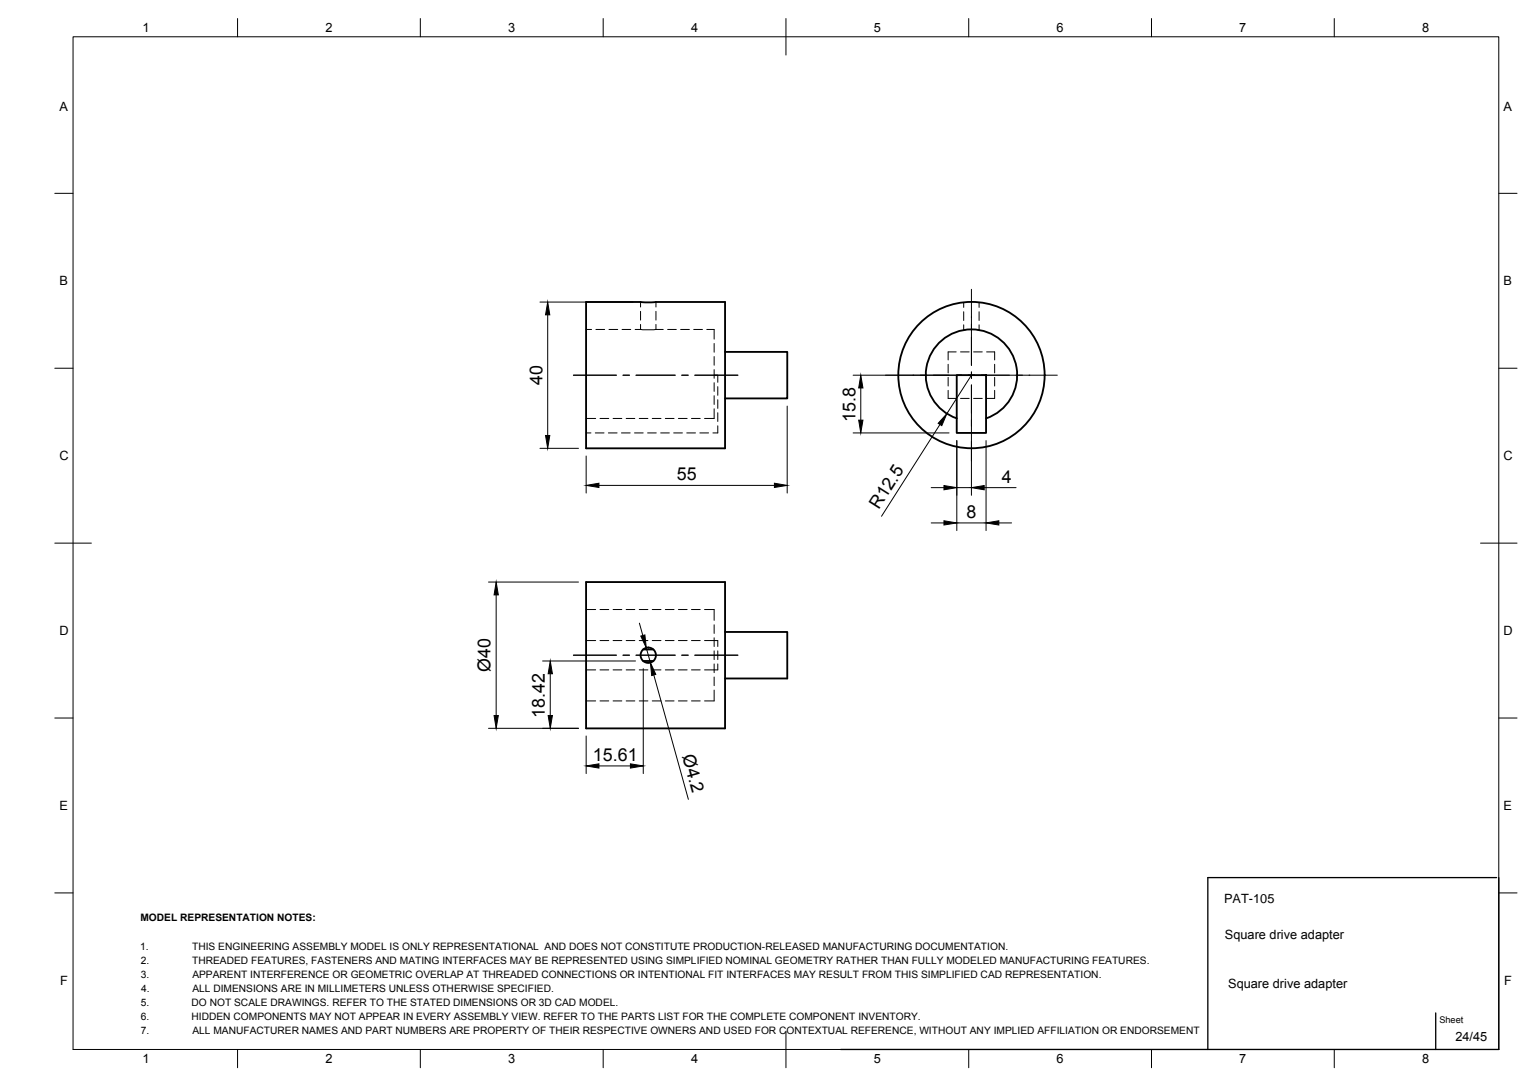
ISO-10303-21;
HEADER;
/* Generated by software containing ST-Developer
 * from STEP Tools, Inc. (www.steptools.com) 
 */

FILE_DESCRIPTION(
/* description */ ('Torque wrench calibration arm'),
/* implementation_level */ '2;1');

FILE_NAME(
/* name */ 'Square drive adapter.step',
/* time_stamp */ '2026-10-28T03:24:52-07:00',
/* author */ (''),
/* organization */ (''),
/* preprocessor_version */ 'ST-DEVELOPER v20.2',
/* originating_system */ 'Autodesk Translation Framework v15.17.0.0',
/* authorisation */ '');

FILE_SCHEMA (('AUTOMOTIVE_DESIGN { 1 0 10303 214 3 1 1 }'));
ENDSEC;

DATA;
#10=MECHANICAL_DESIGN_GEOMETRIC_PRESENTATION_REPRESENTATION('',(#452),#12783);
#267=B_SPLINE_CURVE_WITH_KNOTS('',3,(#11399,#11400,#11401,#11402,#11403,
#11404,#11405,#11406,#11407,#11408,#11409,#11410,#11411,#11412),
 .UNSPECIFIED.,.F.,.F.,(4,2,2,2,2,2,4),(0.779149138325151,0.792661737650614,
0.87192659943798,0.951191461225345,1.03045632301271,1.10972118480008,1.12323378412554),
 .UNSPECIFIED.);
#268=B_SPLINE_CURVE_WITH_KNOTS('',3,(#11418,#11419,#11420,#11421,#11422,
#11423,#11424,#11425,#11426,#11427,#11428,#11429,#11430,#11431,#11432,#11433,
#11434,#11435),.UNSPECIFIED.,.F.,.F.,(4,2,2,2,2,2,2,2,4),(0.,0.0791670250779304,
0.158334050155861,0.237500747381212,0.316667444606564,0.395834141831915,
0.475000839057267,0.554167864135197,0.633334889213128),.UNSPECIFIED.);
#269=B_SPLINE_CURVE_WITH_KNOTS('',3,(#11436,#11437,#11438,#11439,#11440,
#11441,#11442,#11443,#11444,#11445,#11446,#11447,#11448,#11449,#11450,#11451,
#11452,#11453),.UNSPECIFIED.,.F.,.F.,(4,2,2,2,2,2,2,2,4),(0.633334889213128,
0.712501914291058,0.791668939368988,0.87083563659434,0.950002333819691,
1.02916903104504,1.10833572827039,1.18750275334832,1.26666977842626),
 .UNSPECIFIED.);
#270=B_SPLINE_CURVE_WITH_KNOTS('',3,(#11456,#11457,#11458,#11459,#11460,
#11461,#11462,#11463,#11464,#11465,#11466,#11467,#11468,#11469),
 .UNSPECIFIED.,.F.,.F.,(4,2,2,2,2,2,4),(0.145021497508255,0.158534096833718,
0.237798958621083,0.317063820408448,0.396328682195814,0.475593543983179,
0.489106143308642),.UNSPECIFIED.);
#369=SHAPE_REPRESENTATION_RELATIONSHIP('SRR','None',#12952,#406);
#406=ADVANCED_BREP_SHAPE_REPRESENTATION('',(#504),#12761);
#452=STYLED_ITEM('',(#13198),#504);
#504=MANIFOLD_SOLID_BREP('Body1',#6523);
#604=FACE_BOUND('',#1568,.T.);
#605=FACE_BOUND('',#1576,.T.);
#606=FACE_BOUND('',#1578,.T.);
#607=FACE_BOUND('',#1580,.T.);
#770=PLANE('',#7428);
#771=PLANE('',#7433);
#772=PLANE('',#7434);
#773=PLANE('',#7435);
#774=PLANE('',#7436);
#775=PLANE('',#7437);
#776=PLANE('',#7438);
#777=PLANE('',#7439);
#778=PLANE('',#7442);
#779=PLANE('',#7443);
#780=PLANE('',#7444);
#781=PLANE('',#7445);
#782=PLANE('',#7446);
#783=PLANE('',#7447);
#784=PLANE('',#7449);
#1091=FACE_OUTER_BOUND('',#1559,.T.);
#1092=FACE_OUTER_BOUND('',#1560,.T.);
#1093=FACE_OUTER_BOUND('',#1561,.T.);
#1094=FACE_OUTER_BOUND('',#1562,.T.);
#1095=FACE_OUTER_BOUND('',#1563,.T.);
#1096=FACE_OUTER_BOUND('',#1564,.T.);
#1097=FACE_OUTER_BOUND('',#1565,.T.);
#1098=FACE_OUTER_BOUND('',#1566,.T.);
#1099=FACE_OUTER_BOUND('',#1567,.T.);
#1100=FACE_OUTER_BOUND('',#1569,.T.);
#1101=FACE_OUTER_BOUND('',#1570,.T.);
#1102=FACE_OUTER_BOUND('',#1571,.T.);
#1103=FACE_OUTER_BOUND('',#1572,.T.);
#1104=FACE_OUTER_BOUND('',#1573,.T.);
#1105=FACE_OUTER_BOUND('',#1574,.T.);
#1106=FACE_OUTER_BOUND('',#1575,.T.);
#1107=FACE_OUTER_BOUND('',#1577,.T.);
#1108=FACE_OUTER_BOUND('',#1579,.T.);
#1559=EDGE_LOOP('',(#5259,#5260));
#1560=EDGE_LOOP('',(#5261,#5262,#5263,#5264,#5265,#5266,#5267,#5268,#5269));
#1561=EDGE_LOOP('',(#5270,#5271,#5272));
#1562=EDGE_LOOP('',(#5273,#5274,#5275,#5276));
#1563=EDGE_LOOP('',(#5277,#5278,#5279,#5280,#5281,#5282));
#1564=EDGE_LOOP('',(#5283,#5284,#5285,#5286,#5287,#5288));
#1565=EDGE_LOOP('',(#5289,#5290,#5291,#5292));
#1566=EDGE_LOOP('',(#5293,#5294,#5295,#5296));
#1567=EDGE_LOOP('',(#5297));
#1568=EDGE_LOOP('',(#5298,#5299,#5300,#5301));
#1569=EDGE_LOOP('',(#5302,#5303,#5304,#5305));
#1570=EDGE_LOOP('',(#5306,#5307,#5308,#5309));
#1571=EDGE_LOOP('',(#5310,#5311,#5312,#5313));
#1572=EDGE_LOOP('',(#5314,#5315,#5316,#5317));
#1573=EDGE_LOOP('',(#5318,#5319,#5320,#5321));
#1574=EDGE_LOOP('',(#5322,#5323,#5324,#5325));
#1575=EDGE_LOOP('',(#5326));
#1576=EDGE_LOOP('',(#5327,#5328,#5329,#5330));
#1577=EDGE_LOOP('',(#5331,#5332,#5333,#5334));
#1578=EDGE_LOOP('',(#5335,#5336,#5337,#5338));
#1579=EDGE_LOOP('',(#5339,#5340,#5341,#5342));
#1580=EDGE_LOOP('',(#5343,#5344));
#2014=LINE('',#11395,#2429);
#2015=LINE('',#11416,#2430);
#2016=LINE('',#11471,#2431);
#2017=LINE('',#11475,#2432);
#2018=LINE('',#11477,#2433);
#2019=LINE('',#11479,#2434);
#2020=LINE('',#11480,#2435);
#2021=LINE('',#11483,#2436);
#2022=LINE('',#11485,#2437);
#2023=LINE('',#11487,#2438);
#2024=LINE('',#11489,#2439);
#2025=LINE('',#11490,#2440);
#2026=LINE('',#11493,#2441);
#2027=LINE('',#11495,#2442);
#2028=LINE('',#11497,#2443);
#2029=LINE('',#11499,#2444);
#2030=LINE('',#11500,#2445);
#2031=LINE('',#11502,#2446);
#2032=LINE('',#11503,#2447);
#2033=LINE('',#11512,#2448);
#2034=LINE('',#11514,#2449);
#2035=LINE('',#11516,#2450);
#2036=LINE('',#11517,#2451);
#2037=LINE('',#11520,#2452);
#2038=LINE('',#11522,#2453);
#2039=LINE('',#11523,#2454);
#2040=LINE('',#11526,#2455);
#2041=LINE('',#11528,#2456);
#2042=LINE('',#11529,#2457);
#2043=LINE('',#11531,#2458);
#2044=LINE('',#11532,#2459);
#2045=LINE('',#11541,#2460);
#2429=VECTOR('',#8976,1.);
#2430=VECTOR('',#8983,0.21);
#2431=VECTOR('',#8988,1.);
#2432=VECTOR('',#8991,1.);
#2433=VECTOR('',#8992,1.);
#2434=VECTOR('',#8993,1.);
#2435=VECTOR('',#8994,1.);
#2436=VECTOR('',#8997,1.);
#2437=VECTOR('',#8998,1.);
#2438=VECTOR('',#8999,1.);
#2439=VECTOR('',#9000,1.);
#2440=VECTOR('',#9001,1.);
#2441=VECTOR('',#9004,1.);
#2442=VECTOR('',#9005,1.);
#2443=VECTOR('',#9006,1.);
#2444=VECTOR('',#9007,1.);
#2445=VECTOR('',#9008,1.);
#2446=VECTOR('',#9011,1.);
#2447=VECTOR('',#9012,1.);
#2448=VECTOR('',#9023,1.);
#2449=VECTOR('',#9024,1.);
#2450=VECTOR('',#9025,1.);
#2451=VECTOR('',#9026,1.);
#2452=VECTOR('',#9029,1.);
#2453=VECTOR('',#9030,1.);
#2454=VECTOR('',#9031,1.);
#2455=VECTOR('',#9034,1.);
#2456=VECTOR('',#9035,1.);
#2457=VECTOR('',#9036,1.);
#2458=VECTOR('',#9039,1.);
#2459=VECTOR('',#9040,1.);
#2460=VECTOR('',#9055,2.);
#2820=CIRCLE('',#7429,0.21);
#2821=CIRCLE('',#7431,0.21);
#2822=CIRCLE('',#7432,0.21);
#2823=CIRCLE('',#7440,2.);
#2824=CIRCLE('',#7441,1.25);
#2825=CIRCLE('',#7448,1.25);
#2826=CIRCLE('',#7450,2.);
#3282=VERTEX_POINT('',#11393);
#3283=VERTEX_POINT('',#11394);
#3284=VERTEX_POINT('',#11398);
#3285=VERTEX_POINT('',#11413);
#3286=VERTEX_POINT('',#11415);
#3287=VERTEX_POINT('',#11417);
#3288=VERTEX_POINT('',#11454);
#3289=VERTEX_POINT('',#11473);
#3290=VERTEX_POINT('',#11474);
#3291=VERTEX_POINT('',#11476);
#3292=VERTEX_POINT('',#11478);
#3293=VERTEX_POINT('',#11482);
#3294=VERTEX_POINT('',#11484);
#3295=VERTEX_POINT('',#11486);
#3296=VERTEX_POINT('',#11488);
#3297=VERTEX_POINT('',#11492);
#3298=VERTEX_POINT('',#11494);
#3299=VERTEX_POINT('',#11496);
#3300=VERTEX_POINT('',#11498);
#3301=VERTEX_POINT('',#11506);
#3302=VERTEX_POINT('',#11510);
#3303=VERTEX_POINT('',#11511);
#3304=VERTEX_POINT('',#11513);
#3305=VERTEX_POINT('',#11515);
#3306=VERTEX_POINT('',#11519);
#3307=VERTEX_POINT('',#11521);
#3308=VERTEX_POINT('',#11525);
#3309=VERTEX_POINT('',#11527);
#3310=VERTEX_POINT('',#11537);
#3987=EDGE_CURVE('',#3282,#3283,#2014,.T.);
#3988=EDGE_CURVE('',#3282,#3283,#2820,.T.);
#3989=EDGE_CURVE('',#3284,#3282,#267,.T.);
#3990=EDGE_CURVE('',#3285,#3284,#2821,.T.);
#3991=EDGE_CURVE('',#3285,#3286,#2015,.T.);
#3992=EDGE_CURVE('',#3287,#3286,#268,.T.);
#3993=EDGE_CURVE('',#3286,#3287,#269,.T.);
#3994=EDGE_CURVE('',#3288,#3285,#2822,.T.);
#3995=EDGE_CURVE('',#3283,#3288,#270,.T.);
#3996=EDGE_CURVE('',#3288,#3284,#2016,.T.);
#3997=EDGE_CURVE('',#3289,#3290,#2017,.T.);
#3998=EDGE_CURVE('',#3291,#3289,#2018,.T.);
#3999=EDGE_CURVE('',#3291,#3292,#2019,.T.);
#4000=EDGE_CURVE('',#3292,#3290,#2020,.T.);
#4001=EDGE_CURVE('',#3290,#3293,#2021,.T.);
#4002=EDGE_CURVE('',#3292,#3294,#2022,.T.);
#4003=EDGE_CURVE('',#3294,#3295,#2023,.T.);
#4004=EDGE_CURVE('',#3296,#3295,#2024,.T.);
#4005=EDGE_CURVE('',#3293,#3296,#2025,.T.);
#4006=EDGE_CURVE('',#3297,#3289,#2026,.T.);
#4007=EDGE_CURVE('',#3298,#3297,#2027,.T.);
#4008=EDGE_CURVE('',#3299,#3298,#2028,.T.);
#4009=EDGE_CURVE('',#3300,#3299,#2029,.T.);
#4010=EDGE_CURVE('',#3300,#3291,#2030,.T.);
#4011=EDGE_CURVE('',#3295,#3299,#2031,.T.);
#4012=EDGE_CURVE('',#3294,#3300,#2032,.T.);
#4013=EDGE_CURVE('',#3301,#3301,#2823,.T.);
#4014=EDGE_CURVE('',#3293,#3297,#2824,.T.);
#4015=EDGE_CURVE('',#3302,#3303,#2033,.T.);
#4016=EDGE_CURVE('',#3302,#3304,#2034,.T.);
#4017=EDGE_CURVE('',#3305,#3304,#2035,.T.);
#4018=EDGE_CURVE('',#3303,#3305,#2036,.T.);
#4019=EDGE_CURVE('',#3303,#3306,#2037,.T.);
#4020=EDGE_CURVE('',#3307,#3305,#2038,.T.);
#4021=EDGE_CURVE('',#3306,#3307,#2039,.T.);
#4022=EDGE_CURVE('',#3306,#3308,#2040,.T.);
#4023=EDGE_CURVE('',#3309,#3307,#2041,.T.);
#4024=EDGE_CURVE('',#3308,#3309,#2042,.T.);
#4025=EDGE_CURVE('',#3308,#3302,#2043,.T.);
#4026=EDGE_CURVE('',#3304,#3309,#2044,.T.);
#4027=EDGE_CURVE('',#3296,#3298,#2825,.T.);
#4028=EDGE_CURVE('',#3310,#3310,#2826,.T.);
#4029=EDGE_CURVE('',#3301,#3310,#2045,.T.);
#5259=ORIENTED_EDGE('',*,*,#3987,.F.);
#5260=ORIENTED_EDGE('',*,*,#3988,.T.);
#5261=ORIENTED_EDGE('',*,*,#3989,.F.);
#5262=ORIENTED_EDGE('',*,*,#3990,.F.);
#5263=ORIENTED_EDGE('',*,*,#3991,.T.);
#5264=ORIENTED_EDGE('',*,*,#3992,.F.);
#5265=ORIENTED_EDGE('',*,*,#3993,.F.);
#5266=ORIENTED_EDGE('',*,*,#3991,.F.);
#5267=ORIENTED_EDGE('',*,*,#3994,.F.);
#5268=ORIENTED_EDGE('',*,*,#3995,.F.);
#5269=ORIENTED_EDGE('',*,*,#3988,.F.);
#5270=ORIENTED_EDGE('',*,*,#3996,.F.);
#5271=ORIENTED_EDGE('',*,*,#3994,.T.);
#5272=ORIENTED_EDGE('',*,*,#3990,.T.);
#5273=ORIENTED_EDGE('',*,*,#3997,.F.);
#5274=ORIENTED_EDGE('',*,*,#3998,.F.);
#5275=ORIENTED_EDGE('',*,*,#3999,.T.);
#5276=ORIENTED_EDGE('',*,*,#4000,.T.);
#5277=ORIENTED_EDGE('',*,*,#4001,.F.);
#5278=ORIENTED_EDGE('',*,*,#4000,.F.);
#5279=ORIENTED_EDGE('',*,*,#4002,.T.);
#5280=ORIENTED_EDGE('',*,*,#4003,.T.);
#5281=ORIENTED_EDGE('',*,*,#4004,.F.);
#5282=ORIENTED_EDGE('',*,*,#4005,.F.);
#5283=ORIENTED_EDGE('',*,*,#4006,.F.);
#5284=ORIENTED_EDGE('',*,*,#4007,.F.);
#5285=ORIENTED_EDGE('',*,*,#4008,.F.);
#5286=ORIENTED_EDGE('',*,*,#4009,.F.);
#5287=ORIENTED_EDGE('',*,*,#4010,.T.);
#5288=ORIENTED_EDGE('',*,*,#3998,.T.);
#5289=ORIENTED_EDGE('',*,*,#4011,.F.);
#5290=ORIENTED_EDGE('',*,*,#4003,.F.);
#5291=ORIENTED_EDGE('',*,*,#4012,.T.);
#5292=ORIENTED_EDGE('',*,*,#4009,.T.);
#5293=ORIENTED_EDGE('',*,*,#4012,.F.);
#5294=ORIENTED_EDGE('',*,*,#4002,.F.);
#5295=ORIENTED_EDGE('',*,*,#3999,.F.);
#5296=ORIENTED_EDGE('',*,*,#4010,.F.);
#5297=ORIENTED_EDGE('',*,*,#4013,.T.);
#5298=ORIENTED_EDGE('',*,*,#4006,.T.);
#5299=ORIENTED_EDGE('',*,*,#3997,.T.);
#5300=ORIENTED_EDGE('',*,*,#4001,.T.);
#5301=ORIENTED_EDGE('',*,*,#4014,.T.);
#5302=ORIENTED_EDGE('',*,*,#4015,.F.);
#5303=ORIENTED_EDGE('',*,*,#4016,.T.);
#5304=ORIENTED_EDGE('',*,*,#4017,.F.);
#5305=ORIENTED_EDGE('',*,*,#4018,.F.);
#5306=ORIENTED_EDGE('',*,*,#4019,.F.);
#5307=ORIENTED_EDGE('',*,*,#4018,.T.);
#5308=ORIENTED_EDGE('',*,*,#4020,.F.);
#5309=ORIENTED_EDGE('',*,*,#4021,.F.);
#5310=ORIENTED_EDGE('',*,*,#4022,.F.);
#5311=ORIENTED_EDGE('',*,*,#4021,.T.);
#5312=ORIENTED_EDGE('',*,*,#4023,.F.);
#5313=ORIENTED_EDGE('',*,*,#4024,.F.);
#5314=ORIENTED_EDGE('',*,*,#4025,.F.);
#5315=ORIENTED_EDGE('',*,*,#4024,.T.);
#5316=ORIENTED_EDGE('',*,*,#4026,.F.);
#5317=ORIENTED_EDGE('',*,*,#4016,.F.);
#5318=ORIENTED_EDGE('',*,*,#4025,.T.);
#5319=ORIENTED_EDGE('',*,*,#4015,.T.);
#5320=ORIENTED_EDGE('',*,*,#4019,.T.);
#5321=ORIENTED_EDGE('',*,*,#4022,.T.);
#5322=ORIENTED_EDGE('',*,*,#4008,.T.);
#5323=ORIENTED_EDGE('',*,*,#4027,.F.);
#5324=ORIENTED_EDGE('',*,*,#4004,.T.);
#5325=ORIENTED_EDGE('',*,*,#4011,.T.);
#5326=ORIENTED_EDGE('',*,*,#4028,.F.);
#5327=ORIENTED_EDGE('',*,*,#4017,.T.);
#5328=ORIENTED_EDGE('',*,*,#4026,.T.);
#5329=ORIENTED_EDGE('',*,*,#4023,.T.);
#5330=ORIENTED_EDGE('',*,*,#4020,.T.);
#5331=ORIENTED_EDGE('',*,*,#4007,.T.);
#5332=ORIENTED_EDGE('',*,*,#4014,.F.);
#5333=ORIENTED_EDGE('',*,*,#4005,.T.);
#5334=ORIENTED_EDGE('',*,*,#4027,.T.);
#5335=ORIENTED_EDGE('',*,*,#3995,.T.);
#5336=ORIENTED_EDGE('',*,*,#3996,.T.);
#5337=ORIENTED_EDGE('',*,*,#3989,.T.);
#5338=ORIENTED_EDGE('',*,*,#3987,.T.);
#5339=ORIENTED_EDGE('',*,*,#4013,.F.);
#5340=ORIENTED_EDGE('',*,*,#4029,.T.);
#5341=ORIENTED_EDGE('',*,*,#4028,.T.);
#5342=ORIENTED_EDGE('',*,*,#4029,.F.);
#5343=ORIENTED_EDGE('',*,*,#3992,.T.);
#5344=ORIENTED_EDGE('',*,*,#3993,.T.);
#6053=CYLINDRICAL_SURFACE('',#7430,0.21);
#6054=CYLINDRICAL_SURFACE('',#7451,1.25);
#6055=CYLINDRICAL_SURFACE('',#7452,2.);
#6316=ADVANCED_FACE('',(#1091),#770,.T.);
#6317=ADVANCED_FACE('',(#1092),#6053,.F.);
#6318=ADVANCED_FACE('',(#1093),#771,.T.);
#6319=ADVANCED_FACE('',(#1094),#772,.F.);
#6320=ADVANCED_FACE('',(#1095),#773,.F.);
#6321=ADVANCED_FACE('',(#1096),#774,.F.);
#6322=ADVANCED_FACE('',(#1097),#775,.F.);
#6323=ADVANCED_FACE('',(#1098),#776,.T.);
#6324=ADVANCED_FACE('',(#1099,#604),#777,.T.);
#6325=ADVANCED_FACE('',(#1100),#778,.T.);
#6326=ADVANCED_FACE('',(#1101),#779,.T.);
#6327=ADVANCED_FACE('',(#1102),#780,.T.);
#6328=ADVANCED_FACE('',(#1103),#781,.T.);
#6329=ADVANCED_FACE('',(#1104),#782,.F.);
#6330=ADVANCED_FACE('',(#1105),#783,.T.);
#6331=ADVANCED_FACE('',(#1106,#605),#784,.F.);
#6332=ADVANCED_FACE('',(#1107,#606),#6054,.F.);
#6333=ADVANCED_FACE('',(#1108,#607),#6055,.T.);
#6523=CLOSED_SHELL('',(#6316,#6317,#6318,#6319,#6320,#6321,#6322,#6323,
#6324,#6325,#6326,#6327,#6328,#6329,#6330,#6331,#6332,#6333));
#7427=AXIS2_PLACEMENT_3D('',#11391,#8972,#8973);
#7428=AXIS2_PLACEMENT_3D('',#11392,#8974,#8975);
#7429=AXIS2_PLACEMENT_3D('',#11396,#8977,#8978);
#7430=AXIS2_PLACEMENT_3D('',#11397,#8979,#8980);
#7431=AXIS2_PLACEMENT_3D('',#11414,#8981,#8982);
#7432=AXIS2_PLACEMENT_3D('',#11455,#8984,#8985);
#7433=AXIS2_PLACEMENT_3D('',#11470,#8986,#8987);
#7434=AXIS2_PLACEMENT_3D('',#11472,#8989,#8990);
#7435=AXIS2_PLACEMENT_3D('',#11481,#8995,#8996);
#7436=AXIS2_PLACEMENT_3D('',#11491,#9002,#9003);
#7437=AXIS2_PLACEMENT_3D('',#11501,#9009,#9010);
#7438=AXIS2_PLACEMENT_3D('',#11504,#9013,#9014);
#7439=AXIS2_PLACEMENT_3D('',#11505,#9015,#9016);
#7440=AXIS2_PLACEMENT_3D('',#11507,#9017,#9018);
#7441=AXIS2_PLACEMENT_3D('',#11508,#9019,#9020);
#7442=AXIS2_PLACEMENT_3D('',#11509,#9021,#9022);
#7443=AXIS2_PLACEMENT_3D('',#11518,#9027,#9028);
#7444=AXIS2_PLACEMENT_3D('',#11524,#9032,#9033);
#7445=AXIS2_PLACEMENT_3D('',#11530,#9037,#9038);
#7446=AXIS2_PLACEMENT_3D('',#11533,#9041,#9042);
#7447=AXIS2_PLACEMENT_3D('',#11534,#9043,#9044);
#7448=AXIS2_PLACEMENT_3D('',#11535,#9045,#9046);
#7449=AXIS2_PLACEMENT_3D('',#11536,#9047,#9048);
#7450=AXIS2_PLACEMENT_3D('',#11538,#9049,#9050);
#7451=AXIS2_PLACEMENT_3D('',#11539,#9051,#9052);
#7452=AXIS2_PLACEMENT_3D('',#11540,#9053,#9054);
#8972=DIRECTION('axis',(0.,0.,1.));
#8973=DIRECTION('refdir',(1.,0.,0.));
#8974=DIRECTION('center_axis',(0.,0.,1.));
#8975=DIRECTION('ref_axis',(1.,0.,0.));
#8976=DIRECTION('',(0.,1.,0.));
#8977=DIRECTION('center_axis',(0.,0.,1.));
#8978=DIRECTION('ref_axis',(1.,0.,0.));
#8979=DIRECTION('center_axis',(0.,0.,1.));
#8980=DIRECTION('ref_axis',(1.,0.,0.));
#8981=DIRECTION('center_axis',(0.,0.,1.));
#8982=DIRECTION('ref_axis',(1.,0.,0.));
#8983=DIRECTION('',(0.,0.,1.));
#8984=DIRECTION('center_axis',(0.,0.,1.));
#8985=DIRECTION('ref_axis',(1.,0.,0.));
#8986=DIRECTION('center_axis',(0.,0.,1.));
#8987=DIRECTION('ref_axis',(1.,0.,0.));
#8988=DIRECTION('',(0.,-1.,0.));
#8989=DIRECTION('center_axis',(0.,0.,-1.));
#8990=DIRECTION('ref_axis',(-1.,0.,0.));
#8991=DIRECTION('',(1.,0.,0.));
#8992=DIRECTION('',(0.,1.,0.));
#8993=DIRECTION('',(1.,0.,0.));
#8994=DIRECTION('',(0.,1.,0.));
#8995=DIRECTION('center_axis',(1.,0.,0.));
#8996=DIRECTION('ref_axis',(0.,0.,-1.));
#8997=DIRECTION('',(0.,0.,1.));
#8998=DIRECTION('',(0.,0.,1.));
#8999=DIRECTION('',(0.,1.,0.));
#9000=DIRECTION('',(0.,0.,1.));
#9001=DIRECTION('',(0.,-1.,0.));
#9002=DIRECTION('center_axis',(-1.,0.,0.));
#9003=DIRECTION('ref_axis',(0.,0.,1.));
#9004=DIRECTION('',(0.,0.,-1.));
#9005=DIRECTION('',(0.,1.,0.));
#9006=DIRECTION('',(0.,0.,-1.));
#9007=DIRECTION('',(0.,1.,0.));
#9008=DIRECTION('',(0.,0.,-1.));
#9009=DIRECTION('center_axis',(0.,0.,1.));
#9010=DIRECTION('ref_axis',(1.,0.,0.));
#9011=DIRECTION('',(-1.,0.,0.));
#9012=DIRECTION('',(-1.,0.,0.));
#9013=DIRECTION('center_axis',(0.,1.,0.));
#9014=DIRECTION('ref_axis',(1.,0.,0.));
#9015=DIRECTION('center_axis',(0.,1.,0.));
#9016=DIRECTION('ref_axis',(1.,0.,0.));
#9017=DIRECTION('center_axis',(0.,1.,0.));
#9018=DIRECTION('ref_axis',(1.,0.,0.));
#9019=DIRECTION('center_axis',(0.,-1.,0.));
#9020=DIRECTION('ref_axis',(1.,0.,0.));
#9021=DIRECTION('center_axis',(-1.,0.,0.));
#9022=DIRECTION('ref_axis',(0.,0.,1.));
#9023=DIRECTION('',(0.,0.,-1.));
#9024=DIRECTION('',(0.,1.,0.));
#9025=DIRECTION('',(0.,0.,1.));
#9026=DIRECTION('',(0.,1.,0.));
#9027=DIRECTION('center_axis',(0.,0.,-1.));
#9028=DIRECTION('ref_axis',(-1.,0.,0.));
#9029=DIRECTION('',(1.,0.,0.));
#9030=DIRECTION('',(-1.,0.,0.));
#9031=DIRECTION('',(0.,1.,0.));
#9032=DIRECTION('center_axis',(1.,0.,0.));
#9033=DIRECTION('ref_axis',(0.,0.,-1.));
#9034=DIRECTION('',(0.,0.,1.));
#9035=DIRECTION('',(0.,0.,-1.));
#9036=DIRECTION('',(0.,1.,0.));
#9037=DIRECTION('center_axis',(0.,0.,1.));
#9038=DIRECTION('ref_axis',(1.,0.,0.));
#9039=DIRECTION('',(-1.,0.,0.));
#9040=DIRECTION('',(1.,0.,0.));
#9041=DIRECTION('center_axis',(0.,1.,0.));
#9042=DIRECTION('ref_axis',(1.,0.,0.));
#9043=DIRECTION('center_axis',(0.,1.,0.));
#9044=DIRECTION('ref_axis',(1.,0.,0.));
#9045=DIRECTION('center_axis',(0.,-1.,0.));
#9046=DIRECTION('ref_axis',(1.,0.,0.));
#9047=DIRECTION('center_axis',(0.,1.,0.));
#9048=DIRECTION('ref_axis',(1.,0.,0.));
#9049=DIRECTION('center_axis',(0.,1.,0.));
#9050=DIRECTION('ref_axis',(1.,0.,0.));
#9051=DIRECTION('center_axis',(0.,1.,0.));
#9052=DIRECTION('ref_axis',(-1.83697019872103E-16,0.,1.));
#9053=DIRECTION('center_axis',(0.,1.,0.));
#9054=DIRECTION('ref_axis',(1.,0.,0.));
#9055=DIRECTION('',(0.,-1.,0.));
#11391=CARTESIAN_POINT('',(0.,0.,0.));
#11392=CARTESIAN_POINT('Origin',(0.,-2.2,9.24));
#11393=CARTESIAN_POINT('',(0.157797338380593,-2.33856406460551,9.24));
#11394=CARTESIAN_POINT('',(0.157797338380593,-2.06143593539449,9.24));
#11395=CARTESIAN_POINT('',(0.157797338380593,-4.,9.24));
#11396=CARTESIAN_POINT('Origin',(0.,-2.2,9.24));
#11397=CARTESIAN_POINT('Origin',(0.,-2.2,9.24));
#11398=CARTESIAN_POINT('',(-0.157797338380593,-2.33856406460551,9.24));
#11399=CARTESIAN_POINT('Ctrl Pts',(-0.157797338380593,-2.33856406460551,
9.24));
#11400=CARTESIAN_POINT('Ctrl Pts',(-0.154774443077063,-2.34200655046545,
9.24038468131702));
#11401=CARTESIAN_POINT('Ctrl Pts',(-0.151666037725851,-2.3453188103725,
9.24076896680743));
#11402=CARTESIAN_POINT('Ctrl Pts',(-0.129876016991637,-2.36710883110671,
9.24337594943507));
#11403=CARTESIAN_POINT('Ctrl Pts',(-0.1062955610194,-2.38326243211879,9.24574191032087));
#11404=CARTESIAN_POINT('Ctrl Pts',(-0.0545704238568476,-2.4047093901954,
9.24907714823024));
#11405=CARTESIAN_POINT('Ctrl Pts',(-0.0264216205957885,-2.41,9.25));
#11406=CARTESIAN_POINT('Ctrl Pts',(0.0264216205957884,-2.41,9.25));
#11407=CARTESIAN_POINT('Ctrl Pts',(0.0545704238568477,-2.4047093901954,
9.24907714823024));
#11408=CARTESIAN_POINT('Ctrl Pts',(0.106295561019401,-2.38326243211879,
9.24574191032086));
#11409=CARTESIAN_POINT('Ctrl Pts',(0.129876016991637,-2.36710883110671,
9.24337594943507));
#11410=CARTESIAN_POINT('Ctrl Pts',(0.151666037725851,-2.3453188103725,9.24076896680743));
#11411=CARTESIAN_POINT('Ctrl Pts',(0.154774443077063,-2.34200655046545,
9.24038468131702));
#11412=CARTESIAN_POINT('Ctrl Pts',(0.157797338380593,-2.33856406460551,
9.24));
#11413=CARTESIAN_POINT('',(-0.21,-2.2,9.24));
#11414=CARTESIAN_POINT('Origin',(0.,-2.2,9.24));
#11415=CARTESIAN_POINT('',(-0.21,-2.2,9.98894444366855));
#11416=CARTESIAN_POINT('',(-0.21,-2.2,9.24));
#11417=CARTESIAN_POINT('',(0.21,-2.2,9.98894444366855));
#11418=CARTESIAN_POINT('Ctrl Pts',(0.21,-2.2,9.98894444366855));
#11419=CARTESIAN_POINT('Ctrl Pts',(0.21,-2.22638900835931,9.98894444366855));
#11420=CARTESIAN_POINT('Ctrl Pts',(0.204722164681422,-2.25452359377817,
9.98952376620524));
#11421=CARTESIAN_POINT('Ctrl Pts',(0.183284867450471,-2.30625744682115,
9.99161307432363));
#11422=CARTESIAN_POINT('Ctrl Pts',(0.167126466290584,-2.32985838180777,
9.99309254589373));
#11423=CARTESIAN_POINT('Ctrl Pts',(0.129858458976497,-2.36712638912185,
9.99586721250997));
#11424=CARTESIAN_POINT('Ctrl Pts',(0.106257490219278,-2.38328485056549,
9.997343117591));
#11425=CARTESIAN_POINT('Ctrl Pts',(0.0545235237847868,-2.40472219258686,
9.99942425936951));
#11426=CARTESIAN_POINT('Ctrl Pts',(0.0263888990751172,-2.41,10.));
#11427=CARTESIAN_POINT('Ctrl Pts',(-0.0263888990751171,-2.41,10.));
#11428=CARTESIAN_POINT('Ctrl Pts',(-0.0545235237847868,-2.40472219258686,
9.99942425936951));
#11429=CARTESIAN_POINT('Ctrl Pts',(-0.106257490219278,-2.38328485056549,
9.997343117591));
#11430=CARTESIAN_POINT('Ctrl Pts',(-0.129858458976497,-2.36712638912185,
9.99586721250997));
#11431=CARTESIAN_POINT('Ctrl Pts',(-0.167126466290584,-2.32985838180777,
9.99309254589373));
#11432=CARTESIAN_POINT('Ctrl Pts',(-0.183284867450471,-2.30625744682115,
9.99161307432363));
#11433=CARTESIAN_POINT('Ctrl Pts',(-0.204722164681422,-2.25452359377817,
9.98952376620524));
#11434=CARTESIAN_POINT('Ctrl Pts',(-0.21,-2.22638900835931,9.98894444366855));
#11435=CARTESIAN_POINT('Ctrl Pts',(-0.21,-2.2,9.98894444366855));
#11436=CARTESIAN_POINT('Ctrl Pts',(-0.21,-2.2,9.98894444366855));
#11437=CARTESIAN_POINT('Ctrl Pts',(-0.21,-2.17361099164069,9.98894444366855));
#11438=CARTESIAN_POINT('Ctrl Pts',(-0.204722164681422,-2.14547640622183,
9.98952376620524));
#11439=CARTESIAN_POINT('Ctrl Pts',(-0.183284867450471,-2.09374255317885,
9.99161307432363));
#11440=CARTESIAN_POINT('Ctrl Pts',(-0.167126466290584,-2.07014161819223,
9.99309254589373));
#11441=CARTESIAN_POINT('Ctrl Pts',(-0.129858458976497,-2.03287361087815,
9.99586721250997));
#11442=CARTESIAN_POINT('Ctrl Pts',(-0.106257490219278,-2.01671514943451,
9.997343117591));
#11443=CARTESIAN_POINT('Ctrl Pts',(-0.0545235237847867,-1.99527780741314,
9.99942425936951));
#11444=CARTESIAN_POINT('Ctrl Pts',(-0.0263888990751172,-1.99,10.));
#11445=CARTESIAN_POINT('Ctrl Pts',(0.0263888990751171,-1.99,10.));
#11446=CARTESIAN_POINT('Ctrl Pts',(0.0545235237847866,-1.99527780741314,
9.99942425936951));
#11447=CARTESIAN_POINT('Ctrl Pts',(0.106257490219277,-2.01671514943451,
9.997343117591));
#11448=CARTESIAN_POINT('Ctrl Pts',(0.129858458976496,-2.03287361087815,
9.99586721250997));
#11449=CARTESIAN_POINT('Ctrl Pts',(0.167126466290584,-2.07014161819223,
9.99309254589373));
#11450=CARTESIAN_POINT('Ctrl Pts',(0.183284867450471,-2.09374255317885,
9.99161307432363));
#11451=CARTESIAN_POINT('Ctrl Pts',(0.204722164681422,-2.14547640622183,
9.98952376620524));
#11452=CARTESIAN_POINT('Ctrl Pts',(0.21,-2.17361099164069,9.98894444366855));
#11453=CARTESIAN_POINT('Ctrl Pts',(0.21,-2.2,9.98894444366855));
#11454=CARTESIAN_POINT('',(-0.157797338380593,-2.06143593539449,9.24));
#11455=CARTESIAN_POINT('Origin',(0.,-2.2,9.24));
#11456=CARTESIAN_POINT('Ctrl Pts',(0.157797338380593,-2.06143593539449,
9.24));
#11457=CARTESIAN_POINT('Ctrl Pts',(0.154774443077063,-2.05799344953455,
9.24038468131702));
#11458=CARTESIAN_POINT('Ctrl Pts',(0.151666037725851,-2.0546811896275,9.24076896680743));
#11459=CARTESIAN_POINT('Ctrl Pts',(0.129876016991637,-2.03289116889329,
9.24337594943507));
#11460=CARTESIAN_POINT('Ctrl Pts',(0.1062955610194,-2.01673756788121,9.24574191032087));
#11461=CARTESIAN_POINT('Ctrl Pts',(0.0545704238568475,-1.9952906098046,
9.24907714823024));
#11462=CARTESIAN_POINT('Ctrl Pts',(0.0264216205957885,-1.99,9.25));
#11463=CARTESIAN_POINT('Ctrl Pts',(-0.0264216205957884,-1.99,9.25));
#11464=CARTESIAN_POINT('Ctrl Pts',(-0.0545704238568475,-1.9952906098046,
9.24907714823024));
#11465=CARTESIAN_POINT('Ctrl Pts',(-0.1062955610194,-2.01673756788121,9.24574191032087));
#11466=CARTESIAN_POINT('Ctrl Pts',(-0.129876016991637,-2.03289116889329,
9.24337594943507));
#11467=CARTESIAN_POINT('Ctrl Pts',(-0.151666037725851,-2.0546811896275,
9.24076896680743));
#11468=CARTESIAN_POINT('Ctrl Pts',(-0.154774443077063,-2.05799344953455,
9.24038468131702));
#11469=CARTESIAN_POINT('Ctrl Pts',(-0.157797338380593,-2.06143593539449,
9.24));
#11470=CARTESIAN_POINT('Origin',(0.,-2.2,9.24));
#11471=CARTESIAN_POINT('',(-0.157797338380593,-4.,9.24));
#11472=CARTESIAN_POINT('Origin',(0.4,-4.1,6.42));
#11473=CARTESIAN_POINT('',(-0.4,-0.5,6.42));
#11474=CARTESIAN_POINT('',(0.4,-0.5,6.42));
#11475=CARTESIAN_POINT('',(0.2,-0.5,6.42));
#11476=CARTESIAN_POINT('',(-0.4,-4.1,6.42));
#11477=CARTESIAN_POINT('',(-0.4,-4.1,6.42));
#11478=CARTESIAN_POINT('',(0.4,-4.1,6.42));
#11479=CARTESIAN_POINT('',(-0.4,-4.1,6.42));
#11480=CARTESIAN_POINT('',(0.4,-4.1,6.42));
#11481=CARTESIAN_POINT('Origin',(0.4,-4.1,8.));
#11482=CARTESIAN_POINT('',(0.4,-0.5,6.8157280717673));
#11483=CARTESIAN_POINT('',(0.4,-0.5,8.));
#11484=CARTESIAN_POINT('',(0.4,-4.1,8.));
#11485=CARTESIAN_POINT('',(0.4,-4.1,6.42));
#11486=CARTESIAN_POINT('',(0.4,-4.,8.));
#11487=CARTESIAN_POINT('',(0.4,-4.1,8.));
#11488=CARTESIAN_POINT('',(0.4,-4.,6.8157280717673));
#11489=CARTESIAN_POINT('',(0.4,-4.,8.));
#11490=CARTESIAN_POINT('',(0.4,-4.,6.8157280717673));
#11491=CARTESIAN_POINT('Origin',(-0.4,-4.1,6.42));
#11492=CARTESIAN_POINT('',(-0.4,-0.5,6.8157280717673));
#11493=CARTESIAN_POINT('',(-0.4,-0.5,7.21));
#11494=CARTESIAN_POINT('',(-0.4,-4.,6.8157280717673));
#11495=CARTESIAN_POINT('',(-0.4,-4.,6.8157280717673));
#11496=CARTESIAN_POINT('',(-0.4,-4.,8.));
#11497=CARTESIAN_POINT('',(-0.4,-4.,7.21));
#11498=CARTESIAN_POINT('',(-0.4,-4.1,8.));
#11499=CARTESIAN_POINT('',(-0.4,-4.1,8.));
#11500=CARTESIAN_POINT('',(-0.4,-4.1,8.));
#11501=CARTESIAN_POINT('Origin',(-0.4,-4.1,8.));
#11502=CARTESIAN_POINT('',(-0.2,-4.,8.));
#11503=CARTESIAN_POINT('',(0.4,-4.1,8.));
#11504=CARTESIAN_POINT('Origin',(0.,-4.1,7.21));
#11505=CARTESIAN_POINT('Origin',(0.,-0.5,8.));
#11506=CARTESIAN_POINT('',(-2.,-0.5,8.));
#11507=CARTESIAN_POINT('Origin',(0.,-0.5,8.));
#11508=CARTESIAN_POINT('Origin',(0.,-0.5,8.));
#11509=CARTESIAN_POINT('Origin',(-0.635,-6.,7.365));
#11510=CARTESIAN_POINT('',(-0.635,-6.,8.635));
#11511=CARTESIAN_POINT('',(-0.635,-6.,7.365));
#11512=CARTESIAN_POINT('',(-0.635,-6.,8.635));
#11513=CARTESIAN_POINT('',(-0.635,-4.3,8.635));
#11514=CARTESIAN_POINT('',(-0.635,-6.,8.635));
#11515=CARTESIAN_POINT('',(-0.635,-4.3,7.365));
#11516=CARTESIAN_POINT('',(-0.635,-4.3,7.6825));
#11517=CARTESIAN_POINT('',(-0.635,-6.,7.365));
#11518=CARTESIAN_POINT('Origin',(0.635,-6.,7.365));
#11519=CARTESIAN_POINT('',(0.635,-6.,7.365));
#11520=CARTESIAN_POINT('',(-0.635,-6.,7.365));
#11521=CARTESIAN_POINT('',(0.635,-4.3,7.365));
#11522=CARTESIAN_POINT('',(0.3175,-4.3,7.365));
#11523=CARTESIAN_POINT('',(0.635,-6.,7.365));
#11524=CARTESIAN_POINT('Origin',(0.635,-6.,8.635));
#11525=CARTESIAN_POINT('',(0.635,-6.,8.635));
#11526=CARTESIAN_POINT('',(0.635,-6.,7.365));
#11527=CARTESIAN_POINT('',(0.635,-4.3,8.635));
#11528=CARTESIAN_POINT('',(0.635,-4.3,8.3175));
#11529=CARTESIAN_POINT('',(0.635,-6.,8.635));
#11530=CARTESIAN_POINT('Origin',(-0.635,-6.,8.635));
#11531=CARTESIAN_POINT('',(0.635,-6.,8.635));
#11532=CARTESIAN_POINT('',(-0.3175,-4.3,8.635));
#11533=CARTESIAN_POINT('Origin',(0.,-6.,8.));
#11534=CARTESIAN_POINT('Origin',(0.,-4.,8.));
#11535=CARTESIAN_POINT('Origin',(0.,-4.,8.));
#11536=CARTESIAN_POINT('Origin',(0.,-4.3,8.));
#11537=CARTESIAN_POINT('',(-2.,-4.3,8.));
#11538=CARTESIAN_POINT('Origin',(0.,-4.3,8.));
#11539=CARTESIAN_POINT('Origin',(0.,-4.,8.));
#11540=CARTESIAN_POINT('Origin',(0.,-4.,8.));
#11541=CARTESIAN_POINT('',(-2.,-4.,8.));
#12717=UNCERTAINTY_MEASURE_WITH_UNIT(LENGTH_MEASURE(0.001),#12784,
'DISTANCE_ACCURACY_VALUE',
'Maximum model space distance between geometric entities at asserted c
onnectivities');
#12739=UNCERTAINTY_MEASURE_WITH_UNIT(LENGTH_MEASURE(0.001),#12784,
'DISTANCE_ACCURACY_VALUE',
'Maximum model space distance between geometric entities at asserted c
onnectivities');
#12761=(
GEOMETRIC_REPRESENTATION_CONTEXT(3)
GLOBAL_UNCERTAINTY_ASSIGNED_CONTEXT((#12717))
GLOBAL_UNIT_ASSIGNED_CONTEXT((#12784,#12786,#12787))
REPRESENTATION_CONTEXT('','3D')
);
#12783=(
GEOMETRIC_REPRESENTATION_CONTEXT(3)
GLOBAL_UNCERTAINTY_ASSIGNED_CONTEXT((#12739))
GLOBAL_UNIT_ASSIGNED_CONTEXT((#12784,#12786,#12787))
REPRESENTATION_CONTEXT('','3D')
);
#12784=(
LENGTH_UNIT()
NAMED_UNIT(*)
SI_UNIT(.CENTI.,.METRE.)
);
#12786=(
NAMED_UNIT(*)
PLANE_ANGLE_UNIT()
SI_UNIT($,.RADIAN.)
);
#12787=(
NAMED_UNIT(*)
SI_UNIT($,.STERADIAN.)
SOLID_ANGLE_UNIT()
);
#12809=SHAPE_DEFINITION_REPRESENTATION(#12878,#12952);
#12878=PRODUCT_DEFINITION_SHAPE('',$,#12996);
#12952=SHAPE_REPRESENTATION('',(#7427),#12761);
#12974=PRODUCT_DEFINITION_CONTEXT('part definition',#13105,'design');
#12996=PRODUCT_DEFINITION('Square drive adapter','Square drive adapter',
#13039,#12974);
#13039=PRODUCT_DEFINITION_FORMATION('',$,#13128);
#13105=APPLICATION_CONTEXT(
'Core Data for Automotive Mechanical Design Process');
#13106=PRODUCT_CONTEXT('part definition',#13105,'mechanical');
#13128=PRODUCT('Square drive adapter','Square drive adapter',
'Square drive adapter',(#13106));
#13192=COLOUR_RGB('Light Blue',0.38,0.62,0.78);
#13193=FILL_AREA_STYLE_COLOUR('',#13192);
#13194=FILL_AREA_STYLE('',(#13193));
#13195=SURFACE_STYLE_FILL_AREA(#13194);
#13196=SURFACE_SIDE_STYLE('',(#13195));
#13197=SURFACE_STYLE_USAGE(.BOTH.,#13196);
#13198=PRESENTATION_STYLE_ASSIGNMENT((#13197));
ENDSEC;
END-ISO-10303-21;
